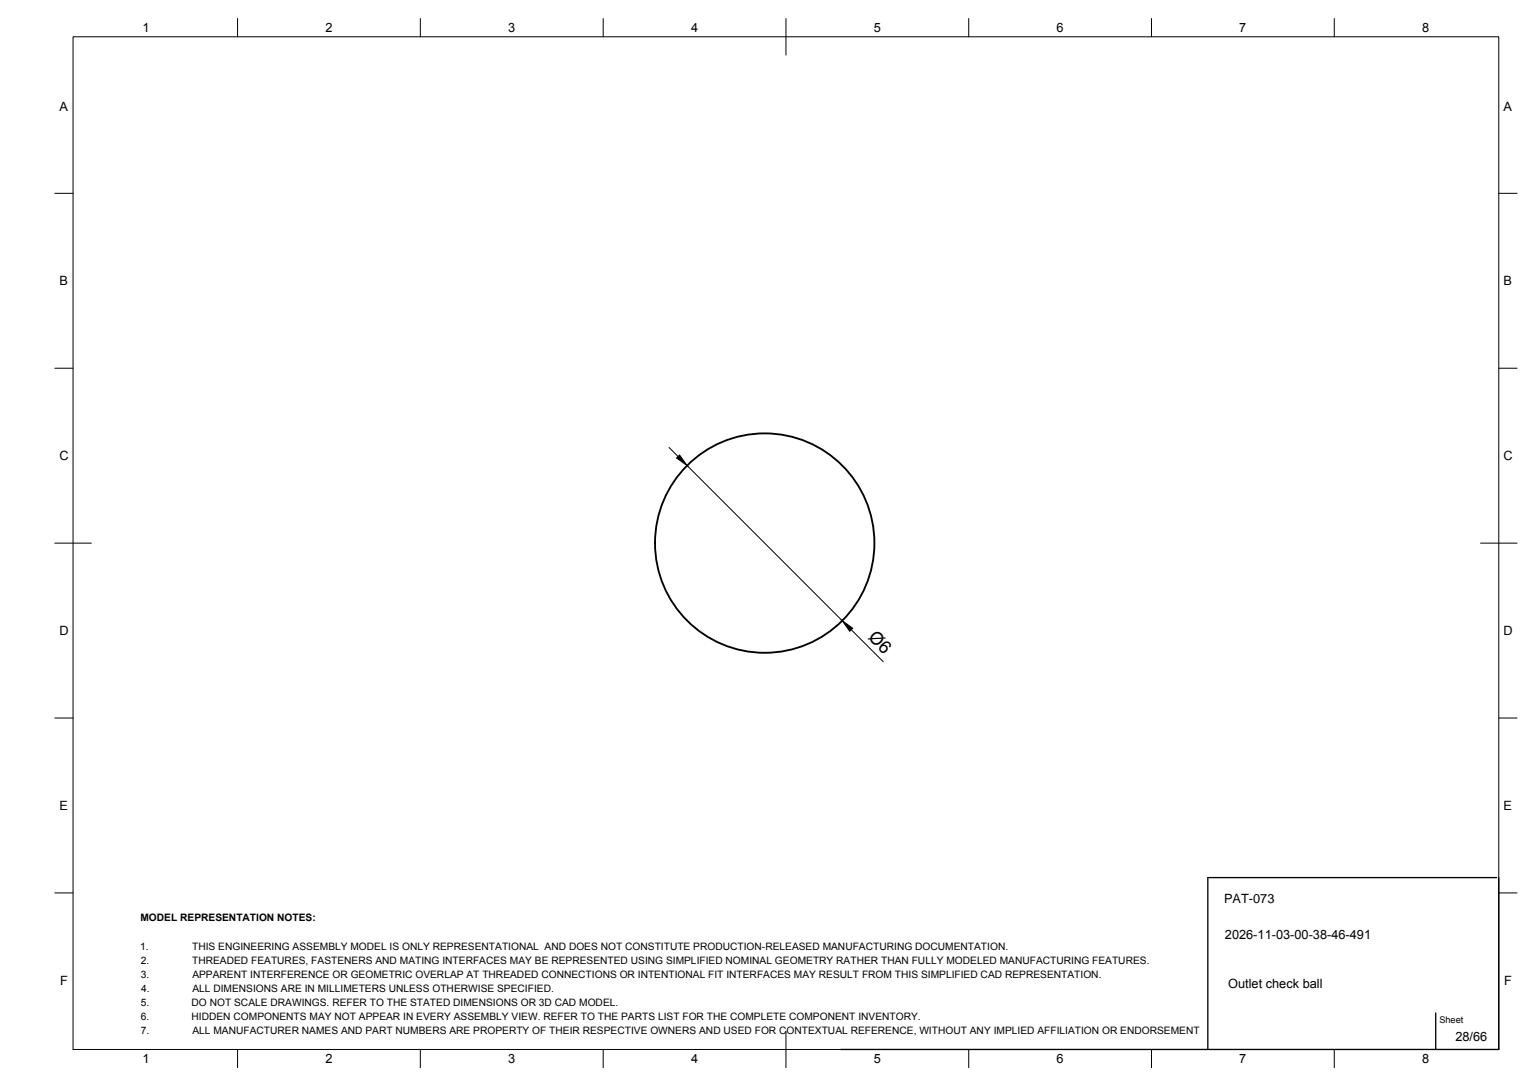
ISO-10303-21;
HEADER;
/* Generated by software containing ST-Developer
 * from STEP Tools, Inc. (www.steptools.com) 
 */

FILE_DESCRIPTION(
/* description */ ('Manual piston pump'),
/* implementation_level */ '2;1');

FILE_NAME(
/* name */ 'Outlet check ball.step',
/* time_stamp */ '2026-11-02T16:54:23-08:00',
/* author */ (''),
/* organization */ (''),
/* preprocessor_version */ 'ST-DEVELOPER v20.2',
/* originating_system */ 'Autodesk Translation Framework v15.17.0.0',
/* authorisation */ '');

FILE_SCHEMA (('AUTOMOTIVE_DESIGN { 1 0 10303 214 3 1 1 }'));
ENDSEC;

DATA;
#10=MECHANICAL_DESIGN_GEOMETRIC_PRESENTATION_REPRESENTATION('',(#730),#19043);
#509=SPHERICAL_SURFACE('',#11004,0.3);
#596=SHAPE_REPRESENTATION_RELATIONSHIP('SRR','None',#19344,#659);
#659=ADVANCED_BREP_SHAPE_REPRESENTATION('',(#800),#19011);
#730=STYLED_ITEM('',(#19661),#800);
#800=MANIFOLD_SOLID_BREP('Body1',#9516);
#1660=FACE_OUTER_BOUND('',#2401,.T.);
#2401=EDGE_LOOP('',(#7791,#7792));
#3004=CIRCLE('',#11005,0.3);
#4866=VERTEX_POINT('',#17273);
#4867=VERTEX_POINT('',#17274);
#5882=EDGE_CURVE('',#4866,#4867,#3004,.T.);
#7791=ORIENTED_EDGE('',*,*,#5882,.T.);
#7792=ORIENTED_EDGE('',*,*,#5882,.F.);
#9265=ADVANCED_FACE('',(#1660),#509,.T.);
#9516=CLOSED_SHELL('',(#9265));
#11003=AXIS2_PLACEMENT_3D('',#17271,#13388,#13389);
#11004=AXIS2_PLACEMENT_3D('',#17272,#13390,#13391);
#11005=AXIS2_PLACEMENT_3D('',#17275,#13392,#13393);
#13388=DIRECTION('axis',(0.,0.,1.));
#13389=DIRECTION('refdir',(1.,0.,0.));
#13390=DIRECTION('center_axis',(0.,0.,1.));
#13391=DIRECTION('ref_axis',(1.,0.,0.));
#13392=DIRECTION('center_axis',(0.,-1.,0.));
#13393=DIRECTION('ref_axis',(-1.,0.,0.));
#17271=CARTESIAN_POINT('',(0.,0.,0.));
#17272=CARTESIAN_POINT('Origin',(1.5,11.4,8.6));
#17273=CARTESIAN_POINT('',(1.5,11.4,8.9));
#17274=CARTESIAN_POINT('',(1.5,11.4,8.3));
#17275=CARTESIAN_POINT('Origin',(1.5,11.4,8.6));
#18940=UNCERTAINTY_MEASURE_WITH_UNIT(LENGTH_MEASURE(0.001),#19044,
'DISTANCE_ACCURACY_VALUE',
'Maximum model space distance between geometric entities at asserted c
onnectivities');
#18972=UNCERTAINTY_MEASURE_WITH_UNIT(LENGTH_MEASURE(0.001),#19044,
'DISTANCE_ACCURACY_VALUE',
'Maximum model space distance between geometric entities at asserted c
onnectivities');
#19011=(
GEOMETRIC_REPRESENTATION_CONTEXT(3)
GLOBAL_UNCERTAINTY_ASSIGNED_CONTEXT((#18940))
GLOBAL_UNIT_ASSIGNED_CONTEXT((#19044,#19046,#19047))
REPRESENTATION_CONTEXT('','3D')
);
#19043=(
GEOMETRIC_REPRESENTATION_CONTEXT(3)
GLOBAL_UNCERTAINTY_ASSIGNED_CONTEXT((#18972))
GLOBAL_UNIT_ASSIGNED_CONTEXT((#19044,#19046,#19047))
REPRESENTATION_CONTEXT('','3D')
);
#19044=(
LENGTH_UNIT()
NAMED_UNIT(*)
SI_UNIT(.CENTI.,.METRE.)
);
#19046=(
NAMED_UNIT(*)
PLANE_ANGLE_UNIT()
SI_UNIT($,.RADIAN.)
);
#19047=(
NAMED_UNIT(*)
SI_UNIT($,.STERADIAN.)
SOLID_ANGLE_UNIT()
);
#19086=SHAPE_DEFINITION_REPRESENTATION(#19163,#19344);
#19163=PRODUCT_DEFINITION_SHAPE('',$,#19415);
#19344=SHAPE_REPRESENTATION('',(#11003),#19011);
#19376=PRODUCT_DEFINITION_CONTEXT('part definition',#19588,'design');
#19415=PRODUCT_DEFINITION('2026-11-03-00-38-46-491','Outlet check ball',
#19485,#19376);
#19485=PRODUCT_DEFINITION_FORMATION('',$,#19628);
#19588=APPLICATION_CONTEXT(
'Core Data for Automotive Mechanical Design Process');
#19589=PRODUCT_CONTEXT('part definition',#19588,'mechanical');
#19628=PRODUCT('2026-11-03-00-38-46-491','Outlet check ball',
'Outlet check ball',(#19589));
#19661=PRESENTATION_STYLE_ASSIGNMENT((#19667));
#19667=SURFACE_STYLE_USAGE(.BOTH.,#19673);
#19673=SURFACE_SIDE_STYLE('',(#19679));
#19679=SURFACE_STYLE_FILL_AREA(#19685);
#19685=FILL_AREA_STYLE('CAD Library Painted - Engineering blue',(#19691));
#19691=FILL_AREA_STYLE_COLOUR('CAD Library Painted - Engineering blue',
#19697);
#19697=COLOUR_RGB('CAD Library Painted - Engineering blue',0.12156862745098,
0.356862745098039,0.6);
ENDSEC;
END-ISO-10303-21;
